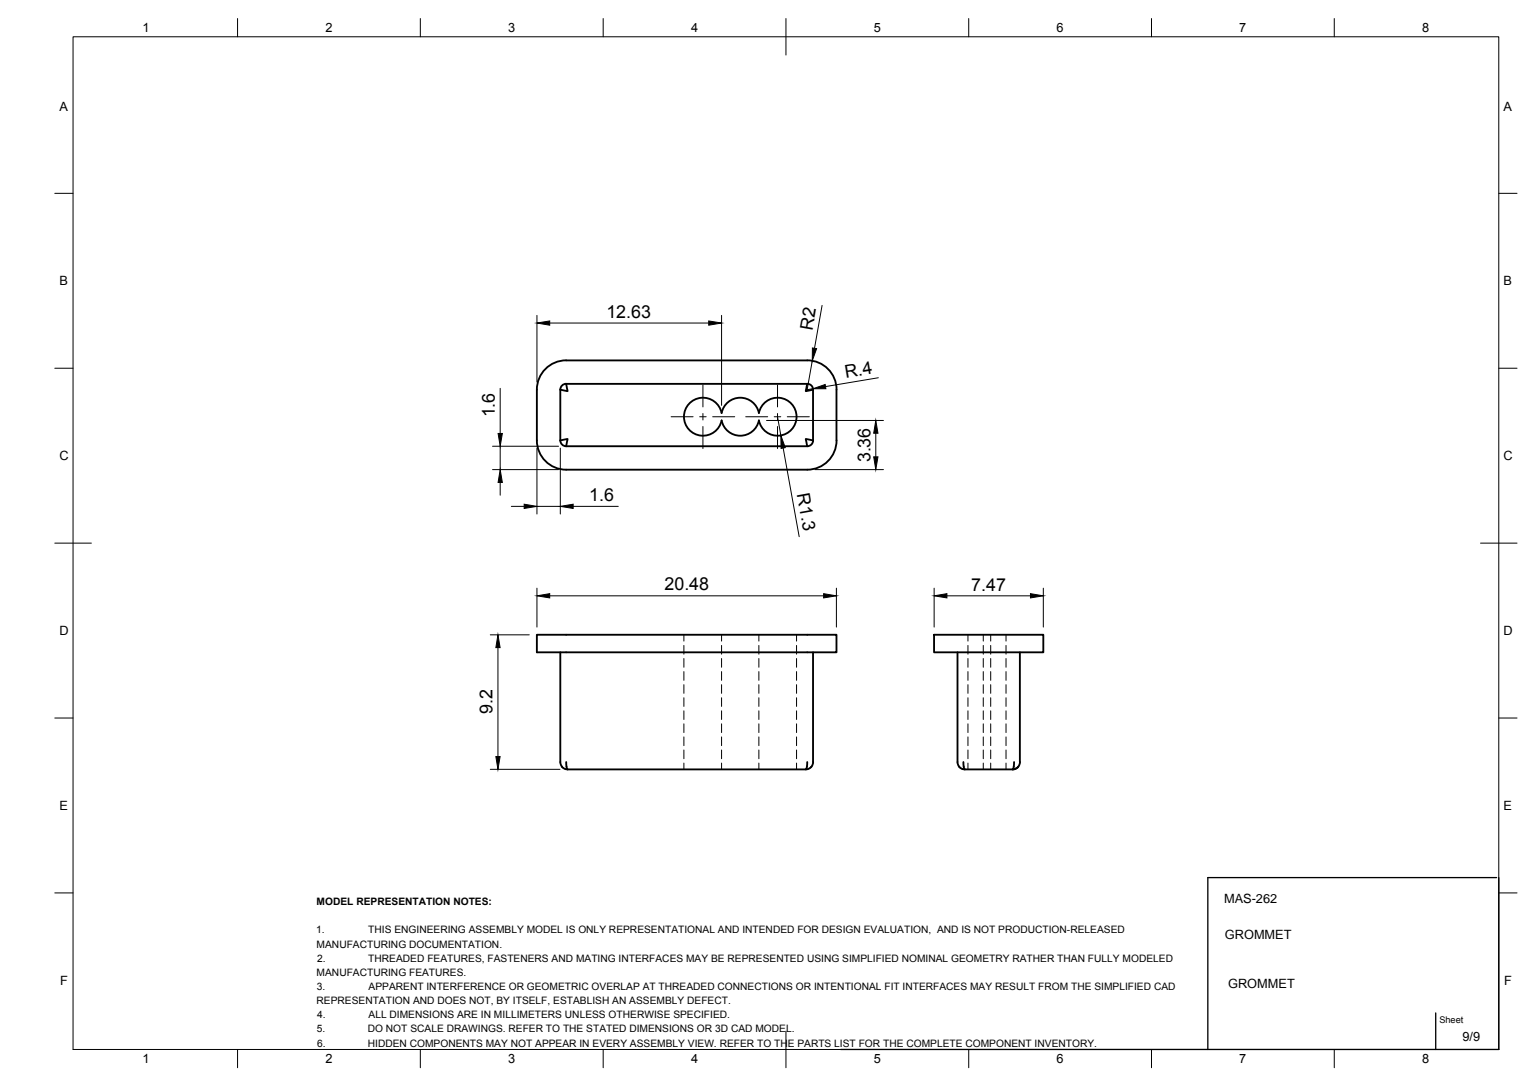
ISO-10303-21;
HEADER;
/* Generated by software containing ST-Developer
 * from STEP Tools, Inc. (www.steptools.com) 
 */

FILE_DESCRIPTION(
/* description */ (''),
/* implementation_level */ '2;1');

FILE_NAME(
/* name */ 'GROMMET.step',
/* time_stamp */ '2026-10-07T02:13:48+06:00',
/* author */ (''),
/* organization */ (''),
/* preprocessor_version */ 'ST-DEVELOPER v20.2',
/* originating_system */ 'Autodesk Translation Framework v15.15.0.0',
/* authorisation */ '');

FILE_SCHEMA (('AUTOMOTIVE_DESIGN { 1 0 10303 214 3 1 1 }'));
ENDSEC;

DATA;
#10=MECHANICAL_DESIGN_GEOMETRIC_PRESENTATION_REPRESENTATION('',(#121),#17042);
#86=B_SPLINE_SURFACE_WITH_KNOTS('',3,3,((#16016,#16017,#16018,#16019,#16020),
(#16021,#16022,#16023,#16024,#16025),(#16026,#16027,#16028,#16029,#16030),
(#16031,#16032,#16033,#16034,#16035),(#16036,#16037,#16038,#16039,#16040)),
 .UNSPECIFIED.,.F.,.F.,.F.,(4,1,4),(4,1,4),(0.,0.5,1.),(0.,0.673198425769241,
1.5707963267949),.UNSPECIFIED.);
#87=B_SPLINE_SURFACE_WITH_KNOTS('',3,3,((#16047,#16048,#16049,#16050,#16051),
(#16052,#16053,#16054,#16055,#16056),(#16057,#16058,#16059,#16060,#16061),
(#16062,#16063,#16064,#16065,#16066),(#16067,#16068,#16069,#16070,#16071)),
 .UNSPECIFIED.,.F.,.F.,.F.,(4,1,4),(4,1,4),(0.,0.5,1.),(1.73472347597681E-16,
0.673198425769242,1.5707963267949),.UNSPECIFIED.);
#88=B_SPLINE_SURFACE_WITH_KNOTS('',3,3,((#16078,#16079,#16080,#16081,#16082),
(#16083,#16084,#16085,#16086,#16087),(#16088,#16089,#16090,#16091,#16092),
(#16093,#16094,#16095,#16096,#16097),(#16098,#16099,#16100,#16101,#16102)),
 .UNSPECIFIED.,.F.,.F.,.F.,(4,1,4),(4,1,4),(0.,0.5,1.),(0.,0.673198425769241,
1.5707963267949),.UNSPECIFIED.);
#89=B_SPLINE_SURFACE_WITH_KNOTS('',3,3,((#16109,#16110,#16111,#16112,#16113),
(#16114,#16115,#16116,#16117,#16118),(#16119,#16120,#16121,#16122,#16123),
(#16124,#16125,#16126,#16127,#16128),(#16129,#16130,#16131,#16132,#16133)),
 .UNSPECIFIED.,.F.,.F.,.F.,(4,1,4),(4,1,4),(0.,0.5,1.),(0.,0.673198425769241,
1.5707963267949),.UNSPECIFIED.);
#97=SHAPE_REPRESENTATION_RELATIONSHIP('SRR','None',#17093,#109);
#109=ADVANCED_BREP_SHAPE_REPRESENTATION('',(#133),#17037);
#121=STYLED_ITEM('',(#17154),#133);
#133=MANIFOLD_SOLID_BREP('Body1',#8122);
#171=FACE_BOUND('',#1345,.T.);
#172=FACE_BOUND('',#1355,.T.);
#173=FACE_BOUND('',#1357,.T.);
#244=ELLIPSE('',#8936,0.509901951359279,0.5);
#245=ELLIPSE('',#8937,0.509901951359279,0.5);
#246=ELLIPSE('',#8939,0.509901951359279,0.5);
#247=ELLIPSE('',#8940,0.509901951359279,0.5);
#248=ELLIPSE('',#8942,0.50990195135928,0.5);
#249=ELLIPSE('',#8943,0.509901951359279,0.5);
#250=ELLIPSE('',#8945,0.509901951359279,0.5);
#251=ELLIPSE('',#8946,0.509901951359279,0.5);
#405=PLANE('',#8952);
#406=PLANE('',#8955);
#407=PLANE('',#8958);
#408=PLANE('',#8963);
#409=PLANE('',#8967);
#410=PLANE('',#8974);
#411=PLANE('',#8978);
#412=PLANE('',#8979);
#413=PLANE('',#8984);
#414=PLANE('',#8991);
#415=PLANE('',#8993);
#822=FACE_OUTER_BOUND('',#1332,.T.);
#823=FACE_OUTER_BOUND('',#1333,.T.);
#824=FACE_OUTER_BOUND('',#1334,.T.);
#825=FACE_OUTER_BOUND('',#1335,.T.);
#826=FACE_OUTER_BOUND('',#1336,.T.);
#827=FACE_OUTER_BOUND('',#1337,.T.);
#828=FACE_OUTER_BOUND('',#1338,.T.);
#829=FACE_OUTER_BOUND('',#1339,.T.);
#830=FACE_OUTER_BOUND('',#1340,.T.);
#831=FACE_OUTER_BOUND('',#1341,.T.);
#832=FACE_OUTER_BOUND('',#1342,.T.);
#833=FACE_OUTER_BOUND('',#1343,.T.);
#834=FACE_OUTER_BOUND('',#1344,.T.);
#835=FACE_OUTER_BOUND('',#1346,.T.);
#836=FACE_OUTER_BOUND('',#1347,.T.);
#837=FACE_OUTER_BOUND('',#1348,.T.);
#838=FACE_OUTER_BOUND('',#1349,.T.);
#839=FACE_OUTER_BOUND('',#1350,.T.);
#840=FACE_OUTER_BOUND('',#1351,.T.);
#841=FACE_OUTER_BOUND('',#1352,.T.);
#842=FACE_OUTER_BOUND('',#1353,.T.);
#843=FACE_OUTER_BOUND('',#1354,.T.);
#844=FACE_OUTER_BOUND('',#1356,.T.);
#845=FACE_OUTER_BOUND('',#1358,.T.);
#846=FACE_OUTER_BOUND('',#1359,.T.);
#847=FACE_OUTER_BOUND('',#1360,.T.);
#848=FACE_OUTER_BOUND('',#1361,.T.);
#849=FACE_OUTER_BOUND('',#1362,.T.);
#850=FACE_OUTER_BOUND('',#1363,.T.);
#851=FACE_OUTER_BOUND('',#1364,.T.);
#852=FACE_OUTER_BOUND('',#1365,.T.);
#1332=EDGE_LOOP('',(#6795,#6796,#6797));
#1333=EDGE_LOOP('',(#6798,#6799,#6800));
#1334=EDGE_LOOP('',(#6801,#6802,#6803));
#1335=EDGE_LOOP('',(#6804,#6805,#6806));
#1336=EDGE_LOOP('',(#6807,#6808,#6809,#6810));
#1337=EDGE_LOOP('',(#6811,#6812,#6813,#6814));
#1338=EDGE_LOOP('',(#6815,#6816,#6817,#6818));
#1339=EDGE_LOOP('',(#6819,#6820,#6821,#6822));
#1340=EDGE_LOOP('',(#6823,#6824,#6825,#6826));
#1341=EDGE_LOOP('',(#6827,#6828,#6829,#6830));
#1342=EDGE_LOOP('',(#6831,#6832,#6833,#6834));
#1343=EDGE_LOOP('',(#6835,#6836,#6837,#6838));
#1344=EDGE_LOOP('',(#6839,#6840,#6841,#6842));
#1345=EDGE_LOOP('',(#6843,#6844,#6845,#6846));
#1346=EDGE_LOOP('',(#6847,#6848,#6849,#6850));
#1347=EDGE_LOOP('',(#6851,#6852,#6853,#6854));
#1348=EDGE_LOOP('',(#6855,#6856,#6857,#6858));
#1349=EDGE_LOOP('',(#6859,#6860,#6861,#6862));
#1350=EDGE_LOOP('',(#6863,#6864,#6865,#6866));
#1351=EDGE_LOOP('',(#6867,#6868,#6869,#6870));
#1352=EDGE_LOOP('',(#6871,#6872,#6873,#6874));
#1353=EDGE_LOOP('',(#6875,#6876,#6877,#6878));
#1354=EDGE_LOOP('',(#6879,#6880,#6881,#6882,#6883,#6884,#6885,#6886));
#1355=EDGE_LOOP('',(#6887,#6888,#6889,#6890));
#1356=EDGE_LOOP('',(#6891,#6892,#6893,#6894,#6895,#6896,#6897,#6898));
#1357=EDGE_LOOP('',(#6899,#6900,#6901,#6902,#6903,#6904,#6905,#6906));
#1358=EDGE_LOOP('',(#6907,#6908,#6909,#6910));
#1359=EDGE_LOOP('',(#6911,#6912,#6913,#6914));
#1360=EDGE_LOOP('',(#6915,#6916,#6917,#6918));
#1361=EDGE_LOOP('',(#6919,#6920,#6921,#6922));
#1362=EDGE_LOOP('',(#6923,#6924,#6925,#6926));
#1363=EDGE_LOOP('',(#6927,#6928,#6929,#6930));
#1364=EDGE_LOOP('',(#6931,#6932,#6933,#6934));
#1365=EDGE_LOOP('',(#6935,#6936,#6937,#6938));
#1818=CIRCLE('',#8938,0.399999999999998);
#1819=CIRCLE('',#8941,0.4);
#1820=CIRCLE('',#8944,0.399999999999997);
#1821=CIRCLE('',#8947,0.4);
#1822=CIRCLE('',#8954,0.399999999999997);
#1823=CIRCLE('',#8957,0.4);
#1824=CIRCLE('',#8959,1.3);
#1825=CIRCLE('',#8960,1.3);
#1826=CIRCLE('',#8961,1.3);
#1827=CIRCLE('',#8962,1.3);
#1828=CIRCLE('',#8965,2.);
#1829=CIRCLE('',#8966,2.);
#1830=CIRCLE('',#8969,2.);
#1831=CIRCLE('',#8970,2.);
#1832=CIRCLE('',#8972,2.);
#1833=CIRCLE('',#8973,2.);
#1834=CIRCLE('',#8976,2.);
#1835=CIRCLE('',#8977,2.);
#1836=CIRCLE('',#8980,1.3);
#1837=CIRCLE('',#8981,1.3);
#1838=CIRCLE('',#8982,1.3);
#1839=CIRCLE('',#8983,1.3);
#1840=CIRCLE('',#8985,0.4);
#1841=CIRCLE('',#8986,0.399999999999998);
#2464=LINE('',#16141,#3042);
#2465=LINE('',#16142,#3043);
#2466=LINE('',#16144,#3044);
#2467=LINE('',#16145,#3045);
#2468=LINE('',#16147,#3046);
#2469=LINE('',#16148,#3047);
#2470=LINE('',#16150,#3048);
#2471=LINE('',#16151,#3049);
#2472=LINE('',#16154,#3050);
#2473=LINE('',#16156,#3051);
#2474=LINE('',#16157,#3052);
#2475=LINE('',#16160,#3053);
#2476=LINE('',#16164,#3054);
#2477=LINE('',#16165,#3055);
#2478=LINE('',#16168,#3056);
#2479=LINE('',#16182,#3057);
#2480=LINE('',#16184,#3058);
#2481=LINE('',#16186,#3059);
#2482=LINE('',#16187,#3060);
#2483=LINE('',#16192,#3061);
#2484=LINE('',#16196,#3062);
#2485=LINE('',#16198,#3063);
#2486=LINE('',#16199,#3064);
#2487=LINE('',#16204,#3065);
#2488=LINE('',#16211,#3066);
#2489=LINE('',#16214,#3067);
#2490=LINE('',#16216,#3068);
#2491=LINE('',#16217,#3069);
#2492=LINE('',#16223,#3070);
#2493=LINE('',#16225,#3071);
#2494=LINE('',#16226,#3072);
#2495=LINE('',#16239,#3073);
#2496=LINE('',#16242,#3074);
#2497=LINE('',#16245,#3075);
#2498=LINE('',#16246,#3076);
#2499=LINE('',#16248,#3077);
#2500=LINE('',#16250,#3078);
#2501=LINE('',#16253,#3079);
#2502=LINE('',#16254,#3080);
#2503=LINE('',#16257,#3081);
#3042=VECTOR('',#11071,20.);
#3043=VECTOR('',#11072,20.);
#3044=VECTOR('',#11075,20.);
#3045=VECTOR('',#11076,20.);
#3046=VECTOR('',#11079,20.);
#3047=VECTOR('',#11080,20.);
#3048=VECTOR('',#11083,20.);
#3049=VECTOR('',#11084,20.);
#3050=VECTOR('',#11087,20.);
#3051=VECTOR('',#11088,20.);
#3052=VECTOR('',#11089,20.);
#3053=VECTOR('',#11092,20.);
#3054=VECTOR('',#11097,20.);
#3055=VECTOR('',#11098,20.);
#3056=VECTOR('',#11101,20.);
#3057=VECTOR('',#11116,20.);
#3058=VECTOR('',#11117,20.);
#3059=VECTOR('',#11118,20.);
#3060=VECTOR('',#11119,20.);
#3061=VECTOR('',#11124,20.);
#3062=VECTOR('',#11129,20.);
#3063=VECTOR('',#11130,20.);
#3064=VECTOR('',#11131,20.);
#3065=VECTOR('',#11136,20.);
#3066=VECTOR('',#11145,20.);
#3067=VECTOR('',#11148,20.);
#3068=VECTOR('',#11149,20.);
#3069=VECTOR('',#11150,20.);
#3070=VECTOR('',#11157,20.);
#3071=VECTOR('',#11160,20.);
#3072=VECTOR('',#11161,20.);
#3073=VECTOR('',#11174,20.);
#3074=VECTOR('',#11177,20.);
#3075=VECTOR('',#11182,20.);
#3076=VECTOR('',#11183,20.);
#3077=VECTOR('',#11186,20.);
#3078=VECTOR('',#11189,20.);
#3079=VECTOR('',#11194,20.);
#3080=VECTOR('',#11195,20.);
#3081=VECTOR('',#11200,20.);
#3704=VERTEX_POINT('',#16041);
#3705=VERTEX_POINT('',#16042);
#3706=VERTEX_POINT('',#16044);
#3707=VERTEX_POINT('',#16072);
#3708=VERTEX_POINT('',#16073);
#3709=VERTEX_POINT('',#16075);
#3710=VERTEX_POINT('',#16103);
#3711=VERTEX_POINT('',#16104);
#3712=VERTEX_POINT('',#16106);
#3713=VERTEX_POINT('',#16134);
#3714=VERTEX_POINT('',#16135);
#3715=VERTEX_POINT('',#16137);
#3716=VERTEX_POINT('',#16153);
#3717=VERTEX_POINT('',#16155);
#3718=VERTEX_POINT('',#16159);
#3719=VERTEX_POINT('',#16163);
#3720=VERTEX_POINT('',#16167);
#3721=VERTEX_POINT('',#16171);
#3722=VERTEX_POINT('',#16172);
#3723=VERTEX_POINT('',#16174);
#3724=VERTEX_POINT('',#16176);
#3725=VERTEX_POINT('',#16180);
#3726=VERTEX_POINT('',#16181);
#3727=VERTEX_POINT('',#16183);
#3728=VERTEX_POINT('',#16185);
#3729=VERTEX_POINT('',#16189);
#3730=VERTEX_POINT('',#16191);
#3731=VERTEX_POINT('',#16195);
#3732=VERTEX_POINT('',#16197);
#3733=VERTEX_POINT('',#16201);
#3734=VERTEX_POINT('',#16203);
#3735=VERTEX_POINT('',#16207);
#3736=VERTEX_POINT('',#16209);
#3737=VERTEX_POINT('',#16213);
#3738=VERTEX_POINT('',#16215);
#3739=VERTEX_POINT('',#16219);
#3740=VERTEX_POINT('',#16221);
#3741=VERTEX_POINT('',#16228);
#3742=VERTEX_POINT('',#16229);
#3743=VERTEX_POINT('',#16231);
#3744=VERTEX_POINT('',#16233);
#3745=VERTEX_POINT('',#16237);
#3746=VERTEX_POINT('',#16238);
#3747=VERTEX_POINT('',#16241);
#4765=EDGE_CURVE('',#3704,#3705,#244,.T.);
#4766=EDGE_CURVE('',#3705,#3706,#245,.T.);
#4767=EDGE_CURVE('',#3706,#3704,#1818,.T.);
#4768=EDGE_CURVE('',#3707,#3708,#246,.T.);
#4769=EDGE_CURVE('',#3708,#3709,#247,.T.);
#4770=EDGE_CURVE('',#3709,#3707,#1819,.T.);
#4771=EDGE_CURVE('',#3710,#3711,#248,.T.);
#4772=EDGE_CURVE('',#3711,#3712,#249,.T.);
#4773=EDGE_CURVE('',#3712,#3710,#1820,.T.);
#4774=EDGE_CURVE('',#3713,#3714,#250,.T.);
#4775=EDGE_CURVE('',#3714,#3715,#251,.T.);
#4776=EDGE_CURVE('',#3715,#3713,#1821,.T.);
#4777=EDGE_CURVE('',#3704,#3715,#2464,.T.);
#4778=EDGE_CURVE('',#3714,#3705,#2465,.T.);
#4779=EDGE_CURVE('',#3711,#3714,#2466,.T.);
#4780=EDGE_CURVE('',#3713,#3712,#2467,.T.);
#4781=EDGE_CURVE('',#3708,#3711,#2468,.T.);
#4782=EDGE_CURVE('',#3710,#3709,#2469,.T.);
#4783=EDGE_CURVE('',#3705,#3708,#2470,.T.);
#4784=EDGE_CURVE('',#3707,#3706,#2471,.T.);
#4785=EDGE_CURVE('',#3716,#3710,#2472,.T.);
#4786=EDGE_CURVE('',#3716,#3717,#2473,.T.);
#4787=EDGE_CURVE('',#3717,#3709,#2474,.T.);
#4788=EDGE_CURVE('',#3718,#3712,#2475,.T.);
#4789=EDGE_CURVE('',#3718,#3716,#1822,.T.);
#4790=EDGE_CURVE('',#3719,#3713,#2476,.T.);
#4791=EDGE_CURVE('',#3719,#3718,#2477,.T.);
#4792=EDGE_CURVE('',#3720,#3715,#2478,.T.);
#4793=EDGE_CURVE('',#3720,#3719,#1823,.T.);
#4794=EDGE_CURVE('',#3721,#3722,#1824,.T.);
#4795=EDGE_CURVE('',#3722,#3723,#1825,.T.);
#4796=EDGE_CURVE('',#3723,#3724,#1826,.T.);
#4797=EDGE_CURVE('',#3724,#3721,#1827,.T.);
#4798=EDGE_CURVE('',#3725,#3726,#2479,.T.);
#4799=EDGE_CURVE('',#3726,#3727,#2480,.T.);
#4800=EDGE_CURVE('',#3728,#3727,#2481,.T.);
#4801=EDGE_CURVE('',#3725,#3728,#2482,.T.);
#4802=EDGE_CURVE('',#3726,#3729,#1828,.T.);
#4803=EDGE_CURVE('',#3729,#3730,#2483,.T.);
#4804=EDGE_CURVE('',#3727,#3730,#1829,.T.);
#4805=EDGE_CURVE('',#3729,#3731,#2484,.T.);
#4806=EDGE_CURVE('',#3731,#3732,#2485,.T.);
#4807=EDGE_CURVE('',#3730,#3732,#2486,.T.);
#4808=EDGE_CURVE('',#3731,#3733,#1830,.T.);
#4809=EDGE_CURVE('',#3733,#3734,#2487,.T.);
#4810=EDGE_CURVE('',#3732,#3734,#1831,.T.);
#4811=EDGE_CURVE('',#3735,#3725,#1832,.T.);
#4812=EDGE_CURVE('',#3736,#3728,#1833,.T.);
#4813=EDGE_CURVE('',#3735,#3736,#2488,.T.);
#4814=EDGE_CURVE('',#3737,#3735,#2489,.T.);
#4815=EDGE_CURVE('',#3738,#3736,#2490,.T.);
#4816=EDGE_CURVE('',#3737,#3738,#2491,.T.);
#4817=EDGE_CURVE('',#3739,#3737,#1834,.T.);
#4818=EDGE_CURVE('',#3740,#3738,#1835,.T.);
#4819=EDGE_CURVE('',#3739,#3740,#2492,.T.);
#4820=EDGE_CURVE('',#3733,#3739,#2493,.T.);
#4821=EDGE_CURVE('',#3734,#3740,#2494,.T.);
#4822=EDGE_CURVE('',#3741,#3742,#1836,.T.);
#4823=EDGE_CURVE('',#3742,#3743,#1837,.T.);
#4824=EDGE_CURVE('',#3743,#3744,#1838,.T.);
#4825=EDGE_CURVE('',#3744,#3741,#1839,.T.);
#4826=EDGE_CURVE('',#3745,#3746,#2495,.T.);
#4827=EDGE_CURVE('',#3717,#3745,#1840,.T.);
#4828=EDGE_CURVE('',#3747,#3720,#2496,.T.);
#4829=EDGE_CURVE('',#3746,#3747,#1841,.T.);
#4830=EDGE_CURVE('',#3721,#3742,#2497,.T.);
#4831=EDGE_CURVE('',#3743,#3724,#2498,.T.);
#4832=EDGE_CURVE('',#3744,#3723,#2499,.T.);
#4833=EDGE_CURVE('',#3741,#3722,#2500,.T.);
#4834=EDGE_CURVE('',#3745,#3707,#2501,.T.);
#4835=EDGE_CURVE('',#3746,#3706,#2502,.T.);
#4836=EDGE_CURVE('',#3747,#3704,#2503,.T.);
#6795=ORIENTED_EDGE('',*,*,#4765,.T.);
#6796=ORIENTED_EDGE('',*,*,#4766,.T.);
#6797=ORIENTED_EDGE('',*,*,#4767,.T.);
#6798=ORIENTED_EDGE('',*,*,#4768,.T.);
#6799=ORIENTED_EDGE('',*,*,#4769,.T.);
#6800=ORIENTED_EDGE('',*,*,#4770,.T.);
#6801=ORIENTED_EDGE('',*,*,#4771,.T.);
#6802=ORIENTED_EDGE('',*,*,#4772,.T.);
#6803=ORIENTED_EDGE('',*,*,#4773,.T.);
#6804=ORIENTED_EDGE('',*,*,#4774,.T.);
#6805=ORIENTED_EDGE('',*,*,#4775,.T.);
#6806=ORIENTED_EDGE('',*,*,#4776,.T.);
#6807=ORIENTED_EDGE('',*,*,#4765,.F.);
#6808=ORIENTED_EDGE('',*,*,#4777,.T.);
#6809=ORIENTED_EDGE('',*,*,#4775,.F.);
#6810=ORIENTED_EDGE('',*,*,#4778,.T.);
#6811=ORIENTED_EDGE('',*,*,#4772,.F.);
#6812=ORIENTED_EDGE('',*,*,#4779,.T.);
#6813=ORIENTED_EDGE('',*,*,#4774,.F.);
#6814=ORIENTED_EDGE('',*,*,#4780,.T.);
#6815=ORIENTED_EDGE('',*,*,#4769,.F.);
#6816=ORIENTED_EDGE('',*,*,#4781,.T.);
#6817=ORIENTED_EDGE('',*,*,#4771,.F.);
#6818=ORIENTED_EDGE('',*,*,#4782,.T.);
#6819=ORIENTED_EDGE('',*,*,#4766,.F.);
#6820=ORIENTED_EDGE('',*,*,#4783,.T.);
#6821=ORIENTED_EDGE('',*,*,#4768,.F.);
#6822=ORIENTED_EDGE('',*,*,#4784,.T.);
#6823=ORIENTED_EDGE('',*,*,#4782,.F.);
#6824=ORIENTED_EDGE('',*,*,#4785,.F.);
#6825=ORIENTED_EDGE('',*,*,#4786,.T.);
#6826=ORIENTED_EDGE('',*,*,#4787,.T.);
#6827=ORIENTED_EDGE('',*,*,#4773,.F.);
#6828=ORIENTED_EDGE('',*,*,#4788,.F.);
#6829=ORIENTED_EDGE('',*,*,#4789,.T.);
#6830=ORIENTED_EDGE('',*,*,#4785,.T.);
#6831=ORIENTED_EDGE('',*,*,#4780,.F.);
#6832=ORIENTED_EDGE('',*,*,#4790,.F.);
#6833=ORIENTED_EDGE('',*,*,#4791,.T.);
#6834=ORIENTED_EDGE('',*,*,#4788,.T.);
#6835=ORIENTED_EDGE('',*,*,#4776,.F.);
#6836=ORIENTED_EDGE('',*,*,#4792,.F.);
#6837=ORIENTED_EDGE('',*,*,#4793,.T.);
#6838=ORIENTED_EDGE('',*,*,#4790,.T.);
#6839=ORIENTED_EDGE('',*,*,#4778,.F.);
#6840=ORIENTED_EDGE('',*,*,#4779,.F.);
#6841=ORIENTED_EDGE('',*,*,#4781,.F.);
#6842=ORIENTED_EDGE('',*,*,#4783,.F.);
#6843=ORIENTED_EDGE('',*,*,#4794,.T.);
#6844=ORIENTED_EDGE('',*,*,#4795,.T.);
#6845=ORIENTED_EDGE('',*,*,#4796,.T.);
#6846=ORIENTED_EDGE('',*,*,#4797,.T.);
#6847=ORIENTED_EDGE('',*,*,#4798,.T.);
#6848=ORIENTED_EDGE('',*,*,#4799,.T.);
#6849=ORIENTED_EDGE('',*,*,#4800,.F.);
#6850=ORIENTED_EDGE('',*,*,#4801,.F.);
#6851=ORIENTED_EDGE('',*,*,#4802,.T.);
#6852=ORIENTED_EDGE('',*,*,#4803,.T.);
#6853=ORIENTED_EDGE('',*,*,#4804,.F.);
#6854=ORIENTED_EDGE('',*,*,#4799,.F.);
#6855=ORIENTED_EDGE('',*,*,#4805,.T.);
#6856=ORIENTED_EDGE('',*,*,#4806,.T.);
#6857=ORIENTED_EDGE('',*,*,#4807,.F.);
#6858=ORIENTED_EDGE('',*,*,#4803,.F.);
#6859=ORIENTED_EDGE('',*,*,#4808,.T.);
#6860=ORIENTED_EDGE('',*,*,#4809,.T.);
#6861=ORIENTED_EDGE('',*,*,#4810,.F.);
#6862=ORIENTED_EDGE('',*,*,#4806,.F.);
#6863=ORIENTED_EDGE('',*,*,#4811,.T.);
#6864=ORIENTED_EDGE('',*,*,#4801,.T.);
#6865=ORIENTED_EDGE('',*,*,#4812,.F.);
#6866=ORIENTED_EDGE('',*,*,#4813,.F.);
#6867=ORIENTED_EDGE('',*,*,#4814,.T.);
#6868=ORIENTED_EDGE('',*,*,#4813,.T.);
#6869=ORIENTED_EDGE('',*,*,#4815,.F.);
#6870=ORIENTED_EDGE('',*,*,#4816,.F.);
#6871=ORIENTED_EDGE('',*,*,#4817,.T.);
#6872=ORIENTED_EDGE('',*,*,#4816,.T.);
#6873=ORIENTED_EDGE('',*,*,#4818,.F.);
#6874=ORIENTED_EDGE('',*,*,#4819,.F.);
#6875=ORIENTED_EDGE('',*,*,#4820,.T.);
#6876=ORIENTED_EDGE('',*,*,#4819,.T.);
#6877=ORIENTED_EDGE('',*,*,#4821,.F.);
#6878=ORIENTED_EDGE('',*,*,#4809,.F.);
#6879=ORIENTED_EDGE('',*,*,#4810,.T.);
#6880=ORIENTED_EDGE('',*,*,#4821,.T.);
#6881=ORIENTED_EDGE('',*,*,#4818,.T.);
#6882=ORIENTED_EDGE('',*,*,#4815,.T.);
#6883=ORIENTED_EDGE('',*,*,#4812,.T.);
#6884=ORIENTED_EDGE('',*,*,#4800,.T.);
#6885=ORIENTED_EDGE('',*,*,#4804,.T.);
#6886=ORIENTED_EDGE('',*,*,#4807,.T.);
#6887=ORIENTED_EDGE('',*,*,#4822,.T.);
#6888=ORIENTED_EDGE('',*,*,#4823,.T.);
#6889=ORIENTED_EDGE('',*,*,#4824,.T.);
#6890=ORIENTED_EDGE('',*,*,#4825,.T.);
#6891=ORIENTED_EDGE('',*,*,#4808,.F.);
#6892=ORIENTED_EDGE('',*,*,#4805,.F.);
#6893=ORIENTED_EDGE('',*,*,#4802,.F.);
#6894=ORIENTED_EDGE('',*,*,#4798,.F.);
#6895=ORIENTED_EDGE('',*,*,#4811,.F.);
#6896=ORIENTED_EDGE('',*,*,#4814,.F.);
#6897=ORIENTED_EDGE('',*,*,#4817,.F.);
#6898=ORIENTED_EDGE('',*,*,#4820,.F.);
#6899=ORIENTED_EDGE('',*,*,#4826,.F.);
#6900=ORIENTED_EDGE('',*,*,#4827,.F.);
#6901=ORIENTED_EDGE('',*,*,#4786,.F.);
#6902=ORIENTED_EDGE('',*,*,#4789,.F.);
#6903=ORIENTED_EDGE('',*,*,#4791,.F.);
#6904=ORIENTED_EDGE('',*,*,#4793,.F.);
#6905=ORIENTED_EDGE('',*,*,#4828,.F.);
#6906=ORIENTED_EDGE('',*,*,#4829,.F.);
#6907=ORIENTED_EDGE('',*,*,#4830,.F.);
#6908=ORIENTED_EDGE('',*,*,#4797,.F.);
#6909=ORIENTED_EDGE('',*,*,#4831,.F.);
#6910=ORIENTED_EDGE('',*,*,#4823,.F.);
#6911=ORIENTED_EDGE('',*,*,#4831,.T.);
#6912=ORIENTED_EDGE('',*,*,#4796,.F.);
#6913=ORIENTED_EDGE('',*,*,#4832,.F.);
#6914=ORIENTED_EDGE('',*,*,#4824,.F.);
#6915=ORIENTED_EDGE('',*,*,#4832,.T.);
#6916=ORIENTED_EDGE('',*,*,#4795,.F.);
#6917=ORIENTED_EDGE('',*,*,#4833,.F.);
#6918=ORIENTED_EDGE('',*,*,#4825,.F.);
#6919=ORIENTED_EDGE('',*,*,#4833,.T.);
#6920=ORIENTED_EDGE('',*,*,#4794,.F.);
#6921=ORIENTED_EDGE('',*,*,#4830,.T.);
#6922=ORIENTED_EDGE('',*,*,#4822,.F.);
#6923=ORIENTED_EDGE('',*,*,#4784,.F.);
#6924=ORIENTED_EDGE('',*,*,#4834,.F.);
#6925=ORIENTED_EDGE('',*,*,#4826,.T.);
#6926=ORIENTED_EDGE('',*,*,#4835,.T.);
#6927=ORIENTED_EDGE('',*,*,#4770,.F.);
#6928=ORIENTED_EDGE('',*,*,#4787,.F.);
#6929=ORIENTED_EDGE('',*,*,#4827,.T.);
#6930=ORIENTED_EDGE('',*,*,#4834,.T.);
#6931=ORIENTED_EDGE('',*,*,#4777,.F.);
#6932=ORIENTED_EDGE('',*,*,#4836,.F.);
#6933=ORIENTED_EDGE('',*,*,#4828,.T.);
#6934=ORIENTED_EDGE('',*,*,#4792,.T.);
#6935=ORIENTED_EDGE('',*,*,#4767,.F.);
#6936=ORIENTED_EDGE('',*,*,#4835,.F.);
#6937=ORIENTED_EDGE('',*,*,#4829,.T.);
#6938=ORIENTED_EDGE('',*,*,#4836,.T.);
#7598=CYLINDRICAL_SURFACE('',#8948,0.5);
#7599=CYLINDRICAL_SURFACE('',#8949,0.5);
#7600=CYLINDRICAL_SURFACE('',#8950,0.5);
#7601=CYLINDRICAL_SURFACE('',#8951,0.5);
#7602=CYLINDRICAL_SURFACE('',#8953,0.399999999999997);
#7603=CYLINDRICAL_SURFACE('',#8956,0.4);
#7604=CYLINDRICAL_SURFACE('',#8964,2.);
#7605=CYLINDRICAL_SURFACE('',#8968,2.);
#7606=CYLINDRICAL_SURFACE('',#8971,2.);
#7607=CYLINDRICAL_SURFACE('',#8975,2.);
#7608=CYLINDRICAL_SURFACE('',#8987,1.3);
#7609=CYLINDRICAL_SURFACE('',#8988,1.3);
#7610=CYLINDRICAL_SURFACE('',#8989,1.3);
#7611=CYLINDRICAL_SURFACE('',#8990,1.3);
#7612=CYLINDRICAL_SURFACE('',#8992,0.4);
#7613=CYLINDRICAL_SURFACE('',#8994,0.399999999999998);
#7984=ADVANCED_FACE('',(#822),#86,.F.);
#7985=ADVANCED_FACE('',(#823),#87,.F.);
#7986=ADVANCED_FACE('',(#824),#88,.F.);
#7987=ADVANCED_FACE('',(#825),#89,.F.);
#7988=ADVANCED_FACE('',(#826),#7598,.T.);
#7989=ADVANCED_FACE('',(#827),#7599,.T.);
#7990=ADVANCED_FACE('',(#828),#7600,.T.);
#7991=ADVANCED_FACE('',(#829),#7601,.T.);
#7992=ADVANCED_FACE('',(#830),#405,.T.);
#7993=ADVANCED_FACE('',(#831),#7602,.T.);
#7994=ADVANCED_FACE('',(#832),#406,.T.);
#7995=ADVANCED_FACE('',(#833),#7603,.T.);
#7996=ADVANCED_FACE('',(#834,#171),#407,.T.);
#7997=ADVANCED_FACE('',(#835),#408,.T.);
#7998=ADVANCED_FACE('',(#836),#7604,.T.);
#7999=ADVANCED_FACE('',(#837),#409,.T.);
#8000=ADVANCED_FACE('',(#838),#7605,.T.);
#8001=ADVANCED_FACE('',(#839),#7606,.T.);
#8002=ADVANCED_FACE('',(#840),#410,.T.);
#8003=ADVANCED_FACE('',(#841),#7607,.T.);
#8004=ADVANCED_FACE('',(#842),#411,.T.);
#8005=ADVANCED_FACE('',(#843,#172),#412,.F.);
#8006=ADVANCED_FACE('',(#844,#173),#413,.T.);
#8007=ADVANCED_FACE('',(#845),#7608,.F.);
#8008=ADVANCED_FACE('',(#846),#7609,.F.);
#8009=ADVANCED_FACE('',(#847),#7610,.F.);
#8010=ADVANCED_FACE('',(#848),#7611,.F.);
#8011=ADVANCED_FACE('',(#849),#414,.T.);
#8012=ADVANCED_FACE('',(#850),#7612,.T.);
#8013=ADVANCED_FACE('',(#851),#415,.T.);
#8014=ADVANCED_FACE('',(#852),#7613,.T.);
#8122=CLOSED_SHELL('',(#7984,#7985,#7986,#7987,#7988,#7989,#7990,#7991,
#7992,#7993,#7994,#7995,#7996,#7997,#7998,#7999,#8000,#8001,#8002,#8003,
#8004,#8005,#8006,#8007,#8008,#8009,#8010,#8011,#8012,#8013,#8014));
#8935=AXIS2_PLACEMENT_3D('',#16015,#11043,#11044);
#8936=AXIS2_PLACEMENT_3D('',#16043,#11045,#11046);
#8937=AXIS2_PLACEMENT_3D('',#16045,#11047,#11048);
#8938=AXIS2_PLACEMENT_3D('',#16046,#11049,#11050);
#8939=AXIS2_PLACEMENT_3D('',#16074,#11051,#11052);
#8940=AXIS2_PLACEMENT_3D('',#16076,#11053,#11054);
#8941=AXIS2_PLACEMENT_3D('',#16077,#11055,#11056);
#8942=AXIS2_PLACEMENT_3D('',#16105,#11057,#11058);
#8943=AXIS2_PLACEMENT_3D('',#16107,#11059,#11060);
#8944=AXIS2_PLACEMENT_3D('',#16108,#11061,#11062);
#8945=AXIS2_PLACEMENT_3D('',#16136,#11063,#11064);
#8946=AXIS2_PLACEMENT_3D('',#16138,#11065,#11066);
#8947=AXIS2_PLACEMENT_3D('',#16139,#11067,#11068);
#8948=AXIS2_PLACEMENT_3D('',#16140,#11069,#11070);
#8949=AXIS2_PLACEMENT_3D('',#16143,#11073,#11074);
#8950=AXIS2_PLACEMENT_3D('',#16146,#11077,#11078);
#8951=AXIS2_PLACEMENT_3D('',#16149,#11081,#11082);
#8952=AXIS2_PLACEMENT_3D('',#16152,#11085,#11086);
#8953=AXIS2_PLACEMENT_3D('',#16158,#11090,#11091);
#8954=AXIS2_PLACEMENT_3D('',#16161,#11093,#11094);
#8955=AXIS2_PLACEMENT_3D('',#16162,#11095,#11096);
#8956=AXIS2_PLACEMENT_3D('',#16166,#11099,#11100);
#8957=AXIS2_PLACEMENT_3D('',#16169,#11102,#11103);
#8958=AXIS2_PLACEMENT_3D('',#16170,#11104,#11105);
#8959=AXIS2_PLACEMENT_3D('',#16173,#11106,#11107);
#8960=AXIS2_PLACEMENT_3D('',#16175,#11108,#11109);
#8961=AXIS2_PLACEMENT_3D('',#16177,#11110,#11111);
#8962=AXIS2_PLACEMENT_3D('',#16178,#11112,#11113);
#8963=AXIS2_PLACEMENT_3D('',#16179,#11114,#11115);
#8964=AXIS2_PLACEMENT_3D('',#16188,#11120,#11121);
#8965=AXIS2_PLACEMENT_3D('',#16190,#11122,#11123);
#8966=AXIS2_PLACEMENT_3D('',#16193,#11125,#11126);
#8967=AXIS2_PLACEMENT_3D('',#16194,#11127,#11128);
#8968=AXIS2_PLACEMENT_3D('',#16200,#11132,#11133);
#8969=AXIS2_PLACEMENT_3D('',#16202,#11134,#11135);
#8970=AXIS2_PLACEMENT_3D('',#16205,#11137,#11138);
#8971=AXIS2_PLACEMENT_3D('',#16206,#11139,#11140);
#8972=AXIS2_PLACEMENT_3D('',#16208,#11141,#11142);
#8973=AXIS2_PLACEMENT_3D('',#16210,#11143,#11144);
#8974=AXIS2_PLACEMENT_3D('',#16212,#11146,#11147);
#8975=AXIS2_PLACEMENT_3D('',#16218,#11151,#11152);
#8976=AXIS2_PLACEMENT_3D('',#16220,#11153,#11154);
#8977=AXIS2_PLACEMENT_3D('',#16222,#11155,#11156);
#8978=AXIS2_PLACEMENT_3D('',#16224,#11158,#11159);
#8979=AXIS2_PLACEMENT_3D('',#16227,#11162,#11163);
#8980=AXIS2_PLACEMENT_3D('',#16230,#11164,#11165);
#8981=AXIS2_PLACEMENT_3D('',#16232,#11166,#11167);
#8982=AXIS2_PLACEMENT_3D('',#16234,#11168,#11169);
#8983=AXIS2_PLACEMENT_3D('',#16235,#11170,#11171);
#8984=AXIS2_PLACEMENT_3D('',#16236,#11172,#11173);
#8985=AXIS2_PLACEMENT_3D('',#16240,#11175,#11176);
#8986=AXIS2_PLACEMENT_3D('',#16243,#11178,#11179);
#8987=AXIS2_PLACEMENT_3D('',#16244,#11180,#11181);
#8988=AXIS2_PLACEMENT_3D('',#16247,#11184,#11185);
#8989=AXIS2_PLACEMENT_3D('',#16249,#11187,#11188);
#8990=AXIS2_PLACEMENT_3D('',#16251,#11190,#11191);
#8991=AXIS2_PLACEMENT_3D('',#16252,#11192,#11193);
#8992=AXIS2_PLACEMENT_3D('',#16255,#11196,#11197);
#8993=AXIS2_PLACEMENT_3D('',#16256,#11198,#11199);
#8994=AXIS2_PLACEMENT_3D('',#16258,#11201,#11202);
#11043=DIRECTION('axis',(0.,0.,1.));
#11044=DIRECTION('refdir',(1.,0.,0.));
#11045=DIRECTION('center_axis',(-0.980580675690919,-0.196116135138188,0.));
#11046=DIRECTION('ref_axis',(-0.196116135138188,0.980580675690919,0.));
#11047=DIRECTION('center_axis',(0.196116135138188,0.980580675690919,0.));
#11048=DIRECTION('ref_axis',(-0.980580675690919,0.196116135138188,0.));
#11049=DIRECTION('center_axis',(0.,0.,-1.));
#11050=DIRECTION('ref_axis',(-1.,0.,0.));
#11051=DIRECTION('center_axis',(0.196116135138184,-0.98058067569092,-2.17732648730911E-15));
#11052=DIRECTION('ref_axis',(-0.98058067569092,-0.196116135138184,0.));
#11053=DIRECTION('center_axis',(-0.980580675690919,0.196116135138188,0.));
#11054=DIRECTION('ref_axis',(-0.196116135138188,-0.980580675690919,0.));
#11055=DIRECTION('center_axis',(0.,0.,-1.));
#11056=DIRECTION('ref_axis',(-2.77555756156289E-15,-1.,0.));
#11057=DIRECTION('center_axis',(0.980580675690919,0.19611613513819,0.));
#11058=DIRECTION('ref_axis',(0.19611613513819,-0.980580675690919,0.));
#11059=DIRECTION('center_axis',(-0.196116135138188,-0.980580675690919,0.));
#11060=DIRECTION('ref_axis',(0.980580675690919,-0.196116135138188,0.));
#11061=DIRECTION('center_axis',(0.,0.,-1.));
#11062=DIRECTION('ref_axis',(1.,0.,0.));
#11063=DIRECTION('center_axis',(-0.196116135138184,0.98058067569092,0.));
#11064=DIRECTION('ref_axis',(0.98058067569092,0.196116135138184,0.));
#11065=DIRECTION('center_axis',(0.98058067569092,-0.196116135138184,0.));
#11066=DIRECTION('ref_axis',(0.196116135138184,0.98058067569092,0.));
#11067=DIRECTION('center_axis',(0.,0.,-1.));
#11068=DIRECTION('ref_axis',(0.,1.,0.));
#11069=DIRECTION('center_axis',(1.,1.34731136305792E-16,4.69378744770455E-33));
#11070=DIRECTION('ref_axis',(0.,0.707106781186546,-0.707106781186549));
#11071=DIRECTION('',(1.,1.34731136305792E-16,4.69378744770455E-33));
#11072=DIRECTION('',(-1.,-1.34731136305792E-16,-4.69378744770455E-33));
#11073=DIRECTION('center_axis',(-1.28138418515522E-15,-1.,-3.48381790312471E-17));
#11074=DIRECTION('ref_axis',(0.707106781186548,0.,-0.707106781186548));
#11075=DIRECTION('',(1.28138418515522E-15,1.,3.48381790312471E-17));
#11076=DIRECTION('',(-1.28138418515522E-15,-1.,-3.48381790312471E-17));
#11077=DIRECTION('center_axis',(-1.,-1.30278772428453E-49,-4.53867519783356E-66));
#11078=DIRECTION('ref_axis',(0.,-0.707106781186549,-0.707106781186546));
#11079=DIRECTION('',(1.,1.30278772428453E-49,4.53867519783356E-66));
#11080=DIRECTION('',(-1.,-1.30278772428453E-49,-4.53867519783356E-66));
#11081=DIRECTION('center_axis',(0.,1.,3.48381790312471E-17));
#11082=DIRECTION('ref_axis',(-0.707106781186548,0.,-0.707106781186548));
#11083=DIRECTION('',(0.,-1.,-3.48381790312471E-17));
#11084=DIRECTION('',(0.,1.,3.48381790312471E-17));
#11085=DIRECTION('center_axis',(1.30278772428453E-49,-1.,0.));
#11086=DIRECTION('ref_axis',(-1.,-1.30278772428453E-49,3.73954024151503E-33));
#11087=DIRECTION('',(0.,0.,-1.));
#11088=DIRECTION('',(-1.,-1.30278772428453E-49,-4.53867519783356E-66));
#11089=DIRECTION('',(0.,0.,-1.));
#11090=DIRECTION('center_axis',(0.,0.,-1.));
#11091=DIRECTION('ref_axis',(1.,5.55111512312582E-15,0.));
#11092=DIRECTION('',(0.,0.,-1.));
#11093=DIRECTION('center_axis',(0.,3.48381790312471E-17,-1.));
#11094=DIRECTION('ref_axis',(1.,5.55111512312582E-15,0.));
#11095=DIRECTION('center_axis',(1.,-1.28138418515522E-15,0.));
#11096=DIRECTION('ref_axis',(-1.28138418515522E-15,-1.,-3.48381790312471E-17));
#11097=DIRECTION('',(0.,0.,-1.));
#11098=DIRECTION('',(-1.28138418515522E-15,-1.,-3.48381790312471E-17));
#11099=DIRECTION('center_axis',(0.,0.,-1.));
#11100=DIRECTION('ref_axis',(-8.32667268468867E-15,1.,0.));
#11101=DIRECTION('',(0.,0.,-1.));
#11102=DIRECTION('center_axis',(0.,3.48381790312471E-17,-1.));
#11103=DIRECTION('ref_axis',(-8.32667268468867E-15,1.,0.));
#11104=DIRECTION('center_axis',(0.,3.48381790312471E-17,-1.));
#11105=DIRECTION('ref_axis',(-1.,0.,0.));
#11106=DIRECTION('center_axis',(0.,-3.48381790312471E-17,1.));
#11107=DIRECTION('ref_axis',(-1.,0.,0.));
#11108=DIRECTION('center_axis',(0.,-3.48381790312471E-17,1.));
#11109=DIRECTION('ref_axis',(-1.,0.,0.));
#11110=DIRECTION('center_axis',(0.,-3.48381790312471E-17,1.));
#11111=DIRECTION('ref_axis',(-1.,0.,0.));
#11112=DIRECTION('center_axis',(0.,-3.48381790312471E-17,1.));
#11113=DIRECTION('ref_axis',(-1.,0.,0.));
#11114=DIRECTION('center_axis',(-1.34731136305792E-16,1.,0.));
#11115=DIRECTION('ref_axis',(-1.,-1.34731136305792E-16,-4.69378744770455E-33));
#11116=DIRECTION('',(-1.,-1.34731136305792E-16,-4.69378744770455E-33));
#11117=DIRECTION('',(0.,0.,1.));
#11118=DIRECTION('',(-1.,-1.34731136305792E-16,-4.69378744770455E-33));
#11119=DIRECTION('',(0.,0.,1.));
#11120=DIRECTION('center_axis',(0.,0.,1.));
#11121=DIRECTION('ref_axis',(-1.,0.,0.));
#11122=DIRECTION('center_axis',(0.,-3.48381790312471E-17,1.));
#11123=DIRECTION('ref_axis',(-1.,0.,0.));
#11124=DIRECTION('',(0.,0.,1.));
#11125=DIRECTION('center_axis',(0.,-3.48381790312471E-17,1.));
#11126=DIRECTION('ref_axis',(-1.,0.,0.));
#11127=DIRECTION('center_axis',(-1.,0.,0.));
#11128=DIRECTION('ref_axis',(0.,-1.,-3.48381790312471E-17));
#11129=DIRECTION('',(0.,-1.,-3.48381790312471E-17));
#11130=DIRECTION('',(0.,0.,1.));
#11131=DIRECTION('',(0.,-1.,-3.48381790312471E-17));
#11132=DIRECTION('center_axis',(0.,0.,1.));
#11133=DIRECTION('ref_axis',(1.66533453693773E-15,-1.,0.));
#11134=DIRECTION('center_axis',(0.,-3.48381790312471E-17,1.));
#11135=DIRECTION('ref_axis',(1.66533453693773E-15,-1.,0.));
#11136=DIRECTION('',(0.,0.,1.));
#11137=DIRECTION('center_axis',(0.,-3.48381790312471E-17,1.));
#11138=DIRECTION('ref_axis',(1.66533453693773E-15,-1.,-3.48381790312471E-17));
#11139=DIRECTION('center_axis',(0.,0.,1.));
#11140=DIRECTION('ref_axis',(-5.55111512312578E-16,1.,0.));
#11141=DIRECTION('center_axis',(0.,-3.48381790312471E-17,1.));
#11142=DIRECTION('ref_axis',(-5.55111512312578E-16,1.,0.));
#11143=DIRECTION('center_axis',(0.,-3.48381790312471E-17,1.));
#11144=DIRECTION('ref_axis',(-5.55111512312578E-16,1.,3.48381790312471E-17));
#11145=DIRECTION('',(0.,0.,1.));
#11146=DIRECTION('center_axis',(1.,-6.40692092577611E-16,0.));
#11147=DIRECTION('ref_axis',(6.40692092577611E-16,1.,3.48381790312471E-17));
#11148=DIRECTION('',(6.40692092577611E-16,1.,3.48381790312471E-17));
#11149=DIRECTION('',(6.40692092577611E-16,1.,3.48381790312471E-17));
#11150=DIRECTION('',(0.,0.,1.));
#11151=DIRECTION('center_axis',(0.,0.,1.));
#11152=DIRECTION('ref_axis',(1.,1.11022302462516E-15,0.));
#11153=DIRECTION('center_axis',(0.,-3.48381790312471E-17,1.));
#11154=DIRECTION('ref_axis',(1.,1.11022302462516E-15,0.));
#11155=DIRECTION('center_axis',(0.,-3.48381790312471E-17,1.));
#11156=DIRECTION('ref_axis',(1.,1.11022302462516E-15,3.86781484965038E-32));
#11157=DIRECTION('',(0.,0.,1.));
#11158=DIRECTION('center_axis',(6.73655681528963E-17,-1.,0.));
#11159=DIRECTION('ref_axis',(1.,6.73655681528963E-17,-1.39264651766275E-33));
#11160=DIRECTION('',(1.,6.73655681528963E-17,2.34689372385228E-33));
#11161=DIRECTION('',(1.,6.73655681528963E-17,-1.39264651766275E-33));
#11162=DIRECTION('center_axis',(0.,3.48381790312471E-17,-1.));
#11163=DIRECTION('ref_axis',(-1.,0.,0.));
#11164=DIRECTION('center_axis',(0.,3.48381790312471E-17,-1.));
#11165=DIRECTION('ref_axis',(-1.,0.,0.));
#11166=DIRECTION('center_axis',(0.,3.48381790312471E-17,-1.));
#11167=DIRECTION('ref_axis',(-1.,0.,0.));
#11168=DIRECTION('center_axis',(0.,3.48381790312471E-17,-1.));
#11169=DIRECTION('ref_axis',(-1.,0.,0.));
#11170=DIRECTION('center_axis',(0.,3.48381790312471E-17,-1.));
#11171=DIRECTION('ref_axis',(-1.,0.,0.));
#11172=DIRECTION('center_axis',(0.,3.48381790312471E-17,-1.));
#11173=DIRECTION('ref_axis',(-1.,0.,0.));
#11174=DIRECTION('',(0.,1.,3.48381790312471E-17));
#11175=DIRECTION('center_axis',(0.,3.48381790312471E-17,-1.));
#11176=DIRECTION('ref_axis',(2.77555756156289E-15,-1.,0.));
#11177=DIRECTION('',(1.,1.34731136305792E-16,4.69378744770455E-33));
#11178=DIRECTION('center_axis',(0.,3.48381790312471E-17,-1.));
#11179=DIRECTION('ref_axis',(-1.,0.,0.));
#11180=DIRECTION('center_axis',(0.,0.,-1.));
#11181=DIRECTION('ref_axis',(1.,1.22464679914735E-16,0.));
#11182=DIRECTION('',(0.,0.,1.));
#11183=DIRECTION('',(0.,0.,-1.));
#11184=DIRECTION('center_axis',(0.,0.,-1.));
#11185=DIRECTION('ref_axis',(-1.,0.,0.));
#11186=DIRECTION('',(0.,0.,-1.));
#11187=DIRECTION('center_axis',(0.,0.,-1.));
#11188=DIRECTION('ref_axis',(-1.,0.,0.));
#11189=DIRECTION('',(0.,0.,-1.));
#11190=DIRECTION('center_axis',(0.,0.,-1.));
#11191=DIRECTION('ref_axis',(-1.,0.,0.));
#11192=DIRECTION('center_axis',(-1.,0.,0.));
#11193=DIRECTION('ref_axis',(0.,1.,3.48381790312471E-17));
#11194=DIRECTION('',(0.,0.,-1.));
#11195=DIRECTION('',(0.,0.,-1.));
#11196=DIRECTION('center_axis',(0.,0.,-1.));
#11197=DIRECTION('ref_axis',(2.77555756156289E-15,-1.,0.));
#11198=DIRECTION('center_axis',(-1.34731136305792E-16,1.,0.));
#11199=DIRECTION('ref_axis',(1.,1.34731136305792E-16,4.69378744770455E-33));
#11200=DIRECTION('',(0.,0.,-1.));
#11201=DIRECTION('center_axis',(0.,0.,-1.));
#11202=DIRECTION('ref_axis',(-1.,0.,0.));
#16015=CARTESIAN_POINT('',(0.,0.,0.));
#16016=CARTESIAN_POINT('Ctrl Pts',(-14.7402854682776,21.6688065021356,-26.5483789742253));
#16017=CARTESIAN_POINT('Ctrl Pts',(-14.7402854682776,21.6688065021356,-26.6605787118535));
#16018=CARTESIAN_POINT('Ctrl Pts',(-14.7220127764577,21.5774430430356,-26.9228448679022));
#16019=CARTESIAN_POINT('Ctrl Pts',(-14.6702053983118,21.3184061523065,-27.0483789742253));
#16020=CARTESIAN_POINT('Ctrl Pts',(-14.6402854682776,21.1688065021356,-27.0483789742253));
#16021=CARTESIAN_POINT('Ctrl Pts',(-14.8450052233973,21.6688065021356,-26.5483789742253));
#16022=CARTESIAN_POINT('Ctrl Pts',(-14.8450052233973,21.6688065021356,-26.6843099042658));
#16023=CARTESIAN_POINT('Ctrl Pts',(-14.779646000333,21.5310977797265,-26.9707326579855));
#16024=CARTESIAN_POINT('Ctrl Pts',(-14.6901520183346,21.2984595322837,-27.0483789742253));
#16025=CARTESIAN_POINT('Ctrl Pts',(-14.6402854682776,21.1688065021356,-27.0483789742253));
#16026=CARTESIAN_POINT('Ctrl Pts',(-15.0535348863446,21.5820559202025,-26.5483789742253));
#16027=CARTESIAN_POINT('Ctrl Pts',(-15.0535348863446,21.5820559202025,-26.7112475141754));
#16028=CARTESIAN_POINT('Ctrl Pts',(-14.8957223019916,21.4242433358495,-27.0209351418812));
#16029=CARTESIAN_POINT('Ctrl Pts',(-14.7300452583802,21.2585662922382,-27.0483789742253));
#16030=CARTESIAN_POINT('Ctrl Pts',(-14.6402854682776,21.1688065021356,-27.0483789742253));
#16031=CARTESIAN_POINT('Ctrl Pts',(-15.1402854682776,21.3735262572552,-26.5483789742253));
#16032=CARTESIAN_POINT('Ctrl Pts',(-15.1402854682776,21.3735262572552,-26.6843099042658));
#16033=CARTESIAN_POINT('Ctrl Pts',(-15.0025767458686,21.308167034191,-26.9707326579855));
#16034=CARTESIAN_POINT('Ctrl Pts',(-14.7699384984258,21.2186730521926,-27.0483789742253));
#16035=CARTESIAN_POINT('Ctrl Pts',(-14.6402854682776,21.1688065021356,-27.0483789742253));
#16036=CARTESIAN_POINT('Ctrl Pts',(-15.1402854682776,21.2688065021356,-26.5483789742253));
#16037=CARTESIAN_POINT('Ctrl Pts',(-15.1402854682776,21.2688065021356,-26.6605787118535));
#16038=CARTESIAN_POINT('Ctrl Pts',(-15.0489220091777,21.2505338103156,-26.9228448679022));
#16039=CARTESIAN_POINT('Ctrl Pts',(-14.7898851184486,21.1987264321698,-27.0483789742253));
#16040=CARTESIAN_POINT('Ctrl Pts',(-14.6402854682776,21.1688065021356,-27.0483789742253));
#16041=CARTESIAN_POINT('',(-14.7402854682776,21.6688065021356,-26.5483789742253));
#16042=CARTESIAN_POINT('',(-14.6402854682776,21.1688065021356,-27.0483789742253));
#16043=CARTESIAN_POINT('Origin',(-14.6402854682776,21.1688065021356,-26.5483789742253));
#16044=CARTESIAN_POINT('',(-15.1402854682776,21.2688065021356,-26.5483789742253));
#16045=CARTESIAN_POINT('Origin',(-14.6402854682776,21.1688065021356,-26.5483789742253));
#16046=CARTESIAN_POINT('Origin',(-14.7402854682776,21.2688065021356,-26.5483789742253));
#16047=CARTESIAN_POINT('Ctrl Pts',(-15.1402854682776,17.8031073387245,-26.5483789742253));
#16048=CARTESIAN_POINT('Ctrl Pts',(-15.1402854682776,17.8031073387245,-26.6605787118535));
#16049=CARTESIAN_POINT('Ctrl Pts',(-15.048928983054,17.8213786357693,-26.9228506801488));
#16050=CARTESIAN_POINT('Ctrl Pts',(-14.7898851184486,17.8731874086903,-27.0483789742253));
#16051=CARTESIAN_POINT('Ctrl Pts',(-14.6402854682776,17.9031073387245,-27.0483789742253));
#16052=CARTESIAN_POINT('Ctrl Pts',(-15.1402854682776,17.6983875836049,-26.5483789742253));
#16053=CARTESIAN_POINT('Ctrl Pts',(-15.1402854682776,17.6983875836049,-26.6843099042658));
#16054=CARTESIAN_POINT('Ctrl Pts',(-15.0025886096795,17.7637448778075,-26.9707646203248));
#16055=CARTESIAN_POINT('Ctrl Pts',(-14.7699384984258,17.8532407886675,-27.0483789742253));
#16056=CARTESIAN_POINT('Ctrl Pts',(-14.6402854682776,17.9031073387245,-27.0483789742253));
#16057=CARTESIAN_POINT('Ctrl Pts',(-15.0535392142239,17.4898535927783,-26.5483789742253));
#16058=CARTESIAN_POINT('Ctrl Pts',(-15.0535392142239,17.4898535927783,-26.7112475141754));
#16059=CARTESIAN_POINT('Ctrl Pts',(-14.8957171704612,17.647675636541,-27.0210148571608));
#16060=CARTESIAN_POINT('Ctrl Pts',(-14.7300452583802,17.813347548622,-27.0483789742253));
#16061=CARTESIAN_POINT('Ctrl Pts',(-14.6402854682777,17.9031073387245,-27.0483789742253));
#16062=CARTESIAN_POINT('Ctrl Pts',(-14.8450052233973,17.4031073387245,-26.5483789742253));
#16063=CARTESIAN_POINT('Ctrl Pts',(-14.8450052233973,17.4031073387245,-26.6843099042658));
#16064=CARTESIAN_POINT('Ctrl Pts',(-14.7796479291947,17.5408041973226,-26.9707646203248));
#16065=CARTESIAN_POINT('Ctrl Pts',(-14.6901520183346,17.7734543085764,-27.0483789742253));
#16066=CARTESIAN_POINT('Ctrl Pts',(-14.6402854682776,17.9031073387245,-27.0483789742253));
#16067=CARTESIAN_POINT('Ctrl Pts',(-14.7402854682776,17.4031073387245,-26.5483789742253));
#16068=CARTESIAN_POINT('Ctrl Pts',(-14.7402854682776,17.4031073387245,-26.6605787118535));
#16069=CARTESIAN_POINT('Ctrl Pts',(-14.7220141712329,17.4944638239482,-26.9228506801488));
#16070=CARTESIAN_POINT('Ctrl Pts',(-14.6702053983118,17.7535076885536,-27.0483789742253));
#16071=CARTESIAN_POINT('Ctrl Pts',(-14.6402854682776,17.9031073387245,-27.0483789742253));
#16072=CARTESIAN_POINT('',(-15.1402854682776,17.8031073387245,-26.5483789742253));
#16073=CARTESIAN_POINT('',(-14.6402854682776,17.9031073387245,-27.0483789742253));
#16074=CARTESIAN_POINT('Origin',(-14.6402854682776,17.9031073387245,-26.5483789742253));
#16075=CARTESIAN_POINT('',(-14.7402854682776,17.4031073387245,-26.5483789742253));
#16076=CARTESIAN_POINT('Origin',(-14.6402854682776,17.9031073387245,-26.5483789742253));
#16077=CARTESIAN_POINT('Origin',(-14.7402854682776,17.8031073387245,-26.5483789742253));
#16078=CARTESIAN_POINT('Ctrl Pts',(1.74028546827765,17.4031073387245,-26.5483789742253));
#16079=CARTESIAN_POINT('Ctrl Pts',(1.74028546827765,17.4031073387245,-26.6605787118535));
#16080=CARTESIAN_POINT('Ctrl Pts',(1.72202043385628,17.4944325108313,-26.9228767774799));
#16081=CARTESIAN_POINT('Ctrl Pts',(1.67020539831183,17.7535076885536,-27.0483789742253));
#16082=CARTESIAN_POINT('Ctrl Pts',(1.64028546827764,17.9031073387245,-27.0483789742253));
#16083=CARTESIAN_POINT('Ctrl Pts',(1.84500522339731,17.4031073387245,-26.5483789742253));
#16084=CARTESIAN_POINT('Ctrl Pts',(1.84500522339731,17.4031073387245,-26.6843099042658));
#16085=CARTESIAN_POINT('Ctrl Pts',(1.77965658989769,17.5407509281098,-26.970908133119));
#16086=CARTESIAN_POINT('Ctrl Pts',(1.69015201833462,17.7734543085764,-27.0483789742253));
#16087=CARTESIAN_POINT('Ctrl Pts',(1.64028546827764,17.9031073387245,-27.0483789742253));
#16088=CARTESIAN_POINT('Ctrl Pts',(2.05355924307323,17.4898335639289,-26.5483789742253));
#16089=CARTESIAN_POINT('Ctrl Pts',(2.05355924307323,17.4898335639289,-26.7112475141754));
#16090=CARTESIAN_POINT('Ctrl Pts',(1.8956931882834,17.6476996187188,-27.0213738612389));
#16091=CARTESIAN_POINT('Ctrl Pts',(1.73004525838021,17.813347548622,-27.0483789742253));
#16092=CARTESIAN_POINT('Ctrl Pts',(1.64028546827764,17.9031073387245,-27.0483789742253));
#16093=CARTESIAN_POINT('Ctrl Pts',(2.14028546827764,17.6983875836049,-26.5483789742253));
#16094=CARTESIAN_POINT('Ctrl Pts',(2.14028546827764,17.6983875836049,-26.6843099042658));
#16095=CARTESIAN_POINT('Ctrl Pts',(2.00264187889234,17.7637362171045,-26.970908133119));
#16096=CARTESIAN_POINT('Ctrl Pts',(1.76993849842579,17.8532407886675,-27.0483789742253));
#16097=CARTESIAN_POINT('Ctrl Pts',(1.64028546827764,17.9031073387245,-27.0483789742253));
#16098=CARTESIAN_POINT('Ctrl Pts',(2.14028546827764,17.8031073387245,-26.5483789742253));
#16099=CARTESIAN_POINT('Ctrl Pts',(2.14028546827764,17.8031073387245,-26.6605787118535));
#16100=CARTESIAN_POINT('Ctrl Pts',(2.04896029617083,17.8213723731459,-26.9228767774799));
#16101=CARTESIAN_POINT('Ctrl Pts',(1.78988511844858,17.8731874086903,-27.0483789742253));
#16102=CARTESIAN_POINT('Ctrl Pts',(1.64028546827764,17.9031073387245,-27.0483789742253));
#16103=CARTESIAN_POINT('',(1.74028546827765,17.4031073387245,-26.5483789742253));
#16104=CARTESIAN_POINT('',(1.64028546827764,17.9031073387245,-27.0483789742253));
#16105=CARTESIAN_POINT('Origin',(1.64028546827764,17.9031073387245,-26.5483789742253));
#16106=CARTESIAN_POINT('',(2.14028546827764,17.8031073387245,-26.5483789742253));
#16107=CARTESIAN_POINT('Origin',(1.64028546827764,17.9031073387245,-26.5483789742253));
#16108=CARTESIAN_POINT('Origin',(1.74028546827765,17.8031073387245,-26.5483789742253));
#16109=CARTESIAN_POINT('Ctrl Pts',(2.14028546827765,21.2688065021356,-26.5483789742253));
#16110=CARTESIAN_POINT('Ctrl Pts',(2.14028546827765,21.2688065021356,-26.6605787118535));
#16111=CARTESIAN_POINT('Ctrl Pts',(2.04895072597714,21.2505395536755,-26.9228688013811));
#16112=CARTESIAN_POINT('Ctrl Pts',(1.78988511844859,21.1987264321698,-27.0483789742253));
#16113=CARTESIAN_POINT('Ctrl Pts',(1.64028546827765,21.1688065021356,-27.0483789742253));
#16114=CARTESIAN_POINT('Ctrl Pts',(2.14028546827765,21.3735262572552,-26.5483789742253));
#16115=CARTESIAN_POINT('Ctrl Pts',(2.14028546827765,21.3735262572552,-26.6843099042658));
#16116=CARTESIAN_POINT('Ctrl Pts',(2.00262559828104,21.3081749767944,-26.9708642714605));
#16117=CARTESIAN_POINT('Ctrl Pts',(1.7699384984258,21.2186730521926,-27.0483789742253));
#16118=CARTESIAN_POINT('Ctrl Pts',(1.64028546827765,21.1688065021356,-27.0483789742253));
#16119=CARTESIAN_POINT('Ctrl Pts',(2.05355301579653,21.5820740496545,-26.5483789742253));
#16120=CARTESIAN_POINT('Ctrl Pts',(2.05355301579653,21.5820740496545,-26.7112475141754));
#16121=CARTESIAN_POINT('Ctrl Pts',(1.8957006850393,21.4242217188972,-27.0212639478808));
#16122=CARTESIAN_POINT('Ctrl Pts',(1.73004525838021,21.2585662922381,-27.0483789742253));
#16123=CARTESIAN_POINT('Ctrl Pts',(1.64028546827765,21.1688065021356,-27.0483789742253));
#16124=CARTESIAN_POINT('Ctrl Pts',(1.84500522339731,21.6688065021356,-26.5483789742253));
#16125=CARTESIAN_POINT('Ctrl Pts',(1.84500522339731,21.6688065021356,-26.6843099042658));
#16126=CARTESIAN_POINT('Ctrl Pts',(1.7796539429365,21.531146632139,-26.9708642714605));
#16127=CARTESIAN_POINT('Ctrl Pts',(1.69015201833463,21.2984595322837,-27.0483789742253));
#16128=CARTESIAN_POINT('Ctrl Pts',(1.64028546827765,21.1688065021356,-27.0483789742253));
#16129=CARTESIAN_POINT('Ctrl Pts',(1.74028546827765,21.6688065021356,-26.5483789742253));
#16130=CARTESIAN_POINT('Ctrl Pts',(1.74028546827765,21.6688065021356,-26.6605787118535));
#16131=CARTESIAN_POINT('Ctrl Pts',(1.72201851981755,21.5774717598351,-26.9228688013811));
#16132=CARTESIAN_POINT('Ctrl Pts',(1.67020539831184,21.3184061523065,-27.0483789742253));
#16133=CARTESIAN_POINT('Ctrl Pts',(1.64028546827765,21.1688065021356,-27.0483789742253));
#16134=CARTESIAN_POINT('',(2.14028546827765,21.2688065021356,-26.5483789742253));
#16135=CARTESIAN_POINT('',(1.64028546827765,21.1688065021356,-27.0483789742253));
#16136=CARTESIAN_POINT('Origin',(1.64028546827765,21.1688065021356,-26.5483789742253));
#16137=CARTESIAN_POINT('',(1.74028546827765,21.6688065021356,-26.5483789742253));
#16138=CARTESIAN_POINT('Origin',(1.64028546827765,21.1688065021356,-26.5483789742253));
#16139=CARTESIAN_POINT('Origin',(1.74028546827765,21.2688065021356,-26.5483789742253));
#16140=CARTESIAN_POINT('Origin',(-10.6201427341388,21.1688065021356,-26.5483789742253));
#16141=CARTESIAN_POINT('',(-10.6201427341388,21.6688065021356,-26.5483789742253));
#16142=CARTESIAN_POINT('',(-10.6201427341388,21.1688065021356,-27.0483789742253));
#16143=CARTESIAN_POINT('Origin',(1.64028546827765,20.4023817112828,-26.5483789742253));
#16144=CARTESIAN_POINT('',(1.64028546827765,20.4023817112828,-27.0483789742253));
#16145=CARTESIAN_POINT('',(2.14028546827765,20.4023817112828,-26.5483789742253));
#16146=CARTESIAN_POINT('Origin',(-2.37985726586118,17.9031073387245,-26.5483789742253));
#16147=CARTESIAN_POINT('',(-2.37985726586118,17.9031073387245,-27.0483789742253));
#16148=CARTESIAN_POINT('',(-2.37985726586118,17.4031073387245,-26.5483789742253));
#16149=CARTESIAN_POINT('Origin',(-14.6402854682776,18.6695321295773,-26.5483789742253));
#16150=CARTESIAN_POINT('',(-14.6402854682776,18.6695321295773,-27.0483789742253));
#16151=CARTESIAN_POINT('',(-15.1402854682776,18.6695321295773,-26.5483789742253));
#16152=CARTESIAN_POINT('Origin',(1.74028546827765,17.4031073387245,-25.0483789742253));
#16153=CARTESIAN_POINT('',(1.74028546827765,17.4031073387245,-19.0483789742253));
#16154=CARTESIAN_POINT('',(1.74028546827765,17.4031073387245,-25.0483789742253));
#16155=CARTESIAN_POINT('',(-14.7402854682776,17.4031073387245,-19.0483789742253));
#16156=CARTESIAN_POINT('',(-2.37985726586118,17.4031073387245,-19.0483789742253));
#16157=CARTESIAN_POINT('',(-14.7402854682776,17.4031073387245,-25.0483789742253));
#16158=CARTESIAN_POINT('Origin',(1.74028546827765,17.8031073387245,-25.0483789742253));
#16159=CARTESIAN_POINT('',(2.14028546827764,17.8031073387245,-19.0483789742253));
#16160=CARTESIAN_POINT('',(2.14028546827764,17.8031073387245,-25.0483789742253));
#16161=CARTESIAN_POINT('Origin',(1.74028546827765,17.8031073387245,-19.0483789742253));
#16162=CARTESIAN_POINT('Origin',(2.14028546827765,21.2688065021356,-25.0483789742253));
#16163=CARTESIAN_POINT('',(2.14028546827765,21.2688065021356,-19.0483789742253));
#16164=CARTESIAN_POINT('',(2.14028546827765,21.2688065021356,-25.0483789742253));
#16165=CARTESIAN_POINT('',(2.14028546827765,20.4023817112828,-19.0483789742253));
#16166=CARTESIAN_POINT('Origin',(1.74028546827765,21.2688065021356,-25.0483789742253));
#16167=CARTESIAN_POINT('',(1.74028546827764,21.6688065021356,-19.0483789742253));
#16168=CARTESIAN_POINT('',(1.74028546827764,21.6688065021356,-25.0483789742253));
#16169=CARTESIAN_POINT('Origin',(1.74028546827765,21.2688065021356,-19.0483789742253));
#16170=CARTESIAN_POINT('Origin',(-6.5,19.5359569204301,-27.0483789742253));
#16171=CARTESIAN_POINT('',(-8.88488236958947,19.6738537403084,-27.0483789742253));
#16172=CARTESIAN_POINT('',(-11.4348823695895,19.6738537403084,-27.0483789742253));
#16173=CARTESIAN_POINT('Origin',(-10.1598823695895,19.4201314511811,-27.0483789742253));
#16174=CARTESIAN_POINT('',(-11.4348823695895,19.1664091620538,-27.0483789742253));
#16175=CARTESIAN_POINT('Origin',(-12.7098823695895,19.4201314511811,-27.0483789742253));
#16176=CARTESIAN_POINT('',(-8.88488236958947,19.1664091620538,-27.0483789742253));
#16177=CARTESIAN_POINT('Origin',(-10.1598823695895,19.4201314511811,-27.0483789742253));
#16178=CARTESIAN_POINT('Origin',(-7.60988236958947,19.4201314511811,-27.0483789742253));
#16179=CARTESIAN_POINT('Origin',(1.74028546827765,23.2688065021356,-25.0483789742253));
#16180=CARTESIAN_POINT('',(1.74028546827765,23.2688065021356,-19.0483789742253));
#16181=CARTESIAN_POINT('',(-14.7402854682776,23.2688065021356,-19.0483789742253));
#16182=CARTESIAN_POINT('',(-2.37985726586118,23.2688065021356,-19.0483789742253));
#16183=CARTESIAN_POINT('',(-14.7402854682776,23.2688065021356,-17.8483789742253));
#16184=CARTESIAN_POINT('',(-14.7402854682776,23.2688065021356,-25.0483789742253));
#16185=CARTESIAN_POINT('',(1.74028546827765,23.2688065021356,-17.8483789742253));
#16186=CARTESIAN_POINT('',(-14.7402854682776,23.2688065021356,-17.8483789742253));
#16187=CARTESIAN_POINT('',(1.74028546827765,23.2688065021356,-25.0483789742253));
#16188=CARTESIAN_POINT('Origin',(-14.7402854682776,21.2688065021356,-25.0483789742253));
#16189=CARTESIAN_POINT('',(-16.7402854682776,21.2688065021356,-19.0483789742253));
#16190=CARTESIAN_POINT('Origin',(-14.7402854682776,21.2688065021356,-19.0483789742253));
#16191=CARTESIAN_POINT('',(-16.7402854682776,21.2688065021356,-17.8483789742253));
#16192=CARTESIAN_POINT('',(-16.7402854682776,21.2688065021356,-25.0483789742253));
#16193=CARTESIAN_POINT('Origin',(-14.7402854682776,21.2688065021356,-17.8483789742253));
#16194=CARTESIAN_POINT('Origin',(-16.7402854682776,21.2688065021356,-25.0483789742253));
#16195=CARTESIAN_POINT('',(-16.7402854682776,17.8031073387245,-19.0483789742253));
#16196=CARTESIAN_POINT('',(-16.7402854682776,20.4023817112828,-19.0483789742253));
#16197=CARTESIAN_POINT('',(-16.7402854682776,17.8031073387245,-17.8483789742253));
#16198=CARTESIAN_POINT('',(-16.7402854682776,17.8031073387245,-25.0483789742253));
#16199=CARTESIAN_POINT('',(-16.7402854682776,17.8031073387245,-17.8483789742253));
#16200=CARTESIAN_POINT('Origin',(-14.7402854682776,17.8031073387245,-25.0483789742253));
#16201=CARTESIAN_POINT('',(-14.7402854682776,15.8031073387245,-19.0483789742253));
#16202=CARTESIAN_POINT('Origin',(-14.7402854682776,17.8031073387245,-19.0483789742253));
#16203=CARTESIAN_POINT('',(-14.7402854682776,15.8031073387245,-17.8483789742253));
#16204=CARTESIAN_POINT('',(-14.7402854682776,15.8031073387245,-25.0483789742253));
#16205=CARTESIAN_POINT('Origin',(-14.7402854682776,17.8031073387245,-17.8483789742253));
#16206=CARTESIAN_POINT('Origin',(1.74028546827765,21.2688065021356,-25.0483789742253));
#16207=CARTESIAN_POINT('',(3.74028546827765,21.2688065021356,-19.0483789742253));
#16208=CARTESIAN_POINT('Origin',(1.74028546827765,21.2688065021356,-19.0483789742253));
#16209=CARTESIAN_POINT('',(3.74028546827765,21.2688065021356,-17.8483789742253));
#16210=CARTESIAN_POINT('Origin',(1.74028546827765,21.2688065021356,-17.8483789742253));
#16211=CARTESIAN_POINT('',(3.74028546827765,21.2688065021356,-25.0483789742253));
#16212=CARTESIAN_POINT('Origin',(3.74028546827765,17.8031073387245,-25.0483789742253));
#16213=CARTESIAN_POINT('',(3.74028546827765,17.8031073387245,-19.0483789742253));
#16214=CARTESIAN_POINT('',(3.74028546827765,18.6695321295773,-19.0483789742253));
#16215=CARTESIAN_POINT('',(3.74028546827765,17.8031073387245,-17.8483789742253));
#16216=CARTESIAN_POINT('',(3.74028546827765,21.2688065021356,-17.8483789742253));
#16217=CARTESIAN_POINT('',(3.74028546827765,17.8031073387245,-25.0483789742253));
#16218=CARTESIAN_POINT('Origin',(1.74028546827765,17.8031073387245,-25.0483789742253));
#16219=CARTESIAN_POINT('',(1.74028546827765,15.8031073387245,-19.0483789742253));
#16220=CARTESIAN_POINT('Origin',(1.74028546827765,17.8031073387245,-19.0483789742253));
#16221=CARTESIAN_POINT('',(1.74028546827765,15.8031073387245,-17.8483789742253));
#16222=CARTESIAN_POINT('Origin',(1.74028546827765,17.8031073387245,-17.8483789742253));
#16223=CARTESIAN_POINT('',(1.74028546827764,15.8031073387245,-25.0483789742253));
#16224=CARTESIAN_POINT('Origin',(-14.7402854682776,15.8031073387245,-25.0483789742253));
#16225=CARTESIAN_POINT('',(-10.6201427341388,15.8031073387245,-19.0483789742253));
#16226=CARTESIAN_POINT('',(1.74028546827764,15.8031073387245,-17.8483789742253));
#16227=CARTESIAN_POINT('Origin',(-6.5,19.5359569204301,-17.8483789742253));
#16228=CARTESIAN_POINT('',(-11.4348823695895,19.6738537403084,-17.8483789742253));
#16229=CARTESIAN_POINT('',(-8.88488236958947,19.6738537403084,-17.8483789742253));
#16230=CARTESIAN_POINT('Origin',(-10.1598823695895,19.4201314511811,-17.8483789742253));
#16231=CARTESIAN_POINT('',(-8.88488236958947,19.1664091620538,-17.8483789742253));
#16232=CARTESIAN_POINT('Origin',(-7.60988236958947,19.4201314511811,-17.8483789742253));
#16233=CARTESIAN_POINT('',(-11.4348823695895,19.1664091620538,-17.8483789742253));
#16234=CARTESIAN_POINT('Origin',(-10.1598823695895,19.4201314511811,-17.8483789742253));
#16235=CARTESIAN_POINT('Origin',(-12.7098823695895,19.4201314511811,-17.8483789742253));
#16236=CARTESIAN_POINT('Origin',(-6.5,19.5359569204301,-19.0483789742253));
#16237=CARTESIAN_POINT('',(-15.1402854682776,17.8031073387245,-19.0483789742253));
#16238=CARTESIAN_POINT('',(-15.1402854682776,21.2688065021356,-19.0483789742253));
#16239=CARTESIAN_POINT('',(-15.1402854682776,18.6695321295773,-19.0483789742253));
#16240=CARTESIAN_POINT('Origin',(-14.7402854682776,17.8031073387245,-19.0483789742253));
#16241=CARTESIAN_POINT('',(-14.7402854682776,21.6688065021356,-19.0483789742253));
#16242=CARTESIAN_POINT('',(-10.6201427341388,21.6688065021356,-19.0483789742253));
#16243=CARTESIAN_POINT('Origin',(-14.7402854682776,21.2688065021356,-19.0483789742253));
#16244=CARTESIAN_POINT('Origin',(-7.60988236958947,19.4201314511811,-25.0483789742253));
#16245=CARTESIAN_POINT('',(-8.88488236958947,19.6738537403084,-25.0483789742253));
#16246=CARTESIAN_POINT('',(-8.88488236958947,19.1664091620538,-25.0483789742253));
#16247=CARTESIAN_POINT('Origin',(-10.1598823695895,19.4201314511811,-25.0483789742253));
#16248=CARTESIAN_POINT('',(-11.4348823695895,19.1664091620538,-25.0483789742253));
#16249=CARTESIAN_POINT('Origin',(-12.7098823695895,19.4201314511811,-25.0483789742253));
#16250=CARTESIAN_POINT('',(-11.4348823695895,19.6738537403084,-25.0483789742253));
#16251=CARTESIAN_POINT('Origin',(-10.1598823695895,19.4201314511811,-25.0483789742253));
#16252=CARTESIAN_POINT('Origin',(-15.1402854682776,17.8031073387245,-25.0483789742253));
#16253=CARTESIAN_POINT('',(-15.1402854682776,17.8031073387245,-25.0483789742253));
#16254=CARTESIAN_POINT('',(-15.1402854682776,21.2688065021356,-25.0483789742253));
#16255=CARTESIAN_POINT('Origin',(-14.7402854682776,17.8031073387245,-25.0483789742253));
#16256=CARTESIAN_POINT('Origin',(-14.7402854682776,21.6688065021356,-25.0483789742253));
#16257=CARTESIAN_POINT('',(-14.7402854682776,21.6688065021356,-25.0483789742253));
#16258=CARTESIAN_POINT('Origin',(-14.7402854682776,21.2688065021356,-25.0483789742253));
#17023=UNCERTAINTY_MEASURE_WITH_UNIT(LENGTH_MEASURE(0.01),#17043,
'DISTANCE_ACCURACY_VALUE',
'Maximum model space distance between geometric entities at asserted c
onnectivities');
#17028=UNCERTAINTY_MEASURE_WITH_UNIT(LENGTH_MEASURE(0.01),#17043,
'DISTANCE_ACCURACY_VALUE',
'Maximum model space distance between geometric entities at asserted c
onnectivities');
#17037=(
GEOMETRIC_REPRESENTATION_CONTEXT(3)
GLOBAL_UNCERTAINTY_ASSIGNED_CONTEXT((#17023))
GLOBAL_UNIT_ASSIGNED_CONTEXT((#17043,#17045,#17046))
REPRESENTATION_CONTEXT('','3D')
);
#17042=(
GEOMETRIC_REPRESENTATION_CONTEXT(3)
GLOBAL_UNCERTAINTY_ASSIGNED_CONTEXT((#17028))
GLOBAL_UNIT_ASSIGNED_CONTEXT((#17043,#17045,#17046))
REPRESENTATION_CONTEXT('','3D')
);
#17043=(
LENGTH_UNIT()
NAMED_UNIT(*)
SI_UNIT(.MILLI.,.METRE.)
);
#17045=(
NAMED_UNIT(*)
PLANE_ANGLE_UNIT()
SI_UNIT($,.RADIAN.)
);
#17046=(
NAMED_UNIT(*)
SI_UNIT($,.STERADIAN.)
SOLID_ANGLE_UNIT()
);
#17055=SHAPE_DEFINITION_REPRESENTATION(#17068,#17093);
#17068=PRODUCT_DEFINITION_SHAPE('',$,#17107);
#17093=SHAPE_REPRESENTATION('',(#8935),#17037);
#17098=PRODUCT_DEFINITION_CONTEXT('part definition',#17139,'design');
#17107=PRODUCT_DEFINITION('GROMMET','GROMMET',#17120,#17098);
#17120=PRODUCT_DEFINITION_FORMATION('',$,#17149);
#17139=APPLICATION_CONTEXT(
'Core Data for Automotive Mechanical Design Process');
#17140=PRODUCT_CONTEXT('part definition',#17139,'mechanical');
#17149=PRODUCT('GROMMET','GROMMET',$,(#17140));
#17154=PRESENTATION_STYLE_ASSIGNMENT((#17155));
#17155=SURFACE_STYLE_USAGE(.BOTH.,#17156);
#17156=SURFACE_SIDE_STYLE('',(#17157));
#17157=SURFACE_STYLE_FILL_AREA(#17158);
#17158=FILL_AREA_STYLE('Steel - Satin',(#17159));
#17159=FILL_AREA_STYLE_COLOUR('Steel - Satin',#17160);
#17160=COLOUR_RGB('Steel - Satin', 0.09019608, 0.27058824, 0.51372549);
ENDSEC;
END-ISO-10303-21;
